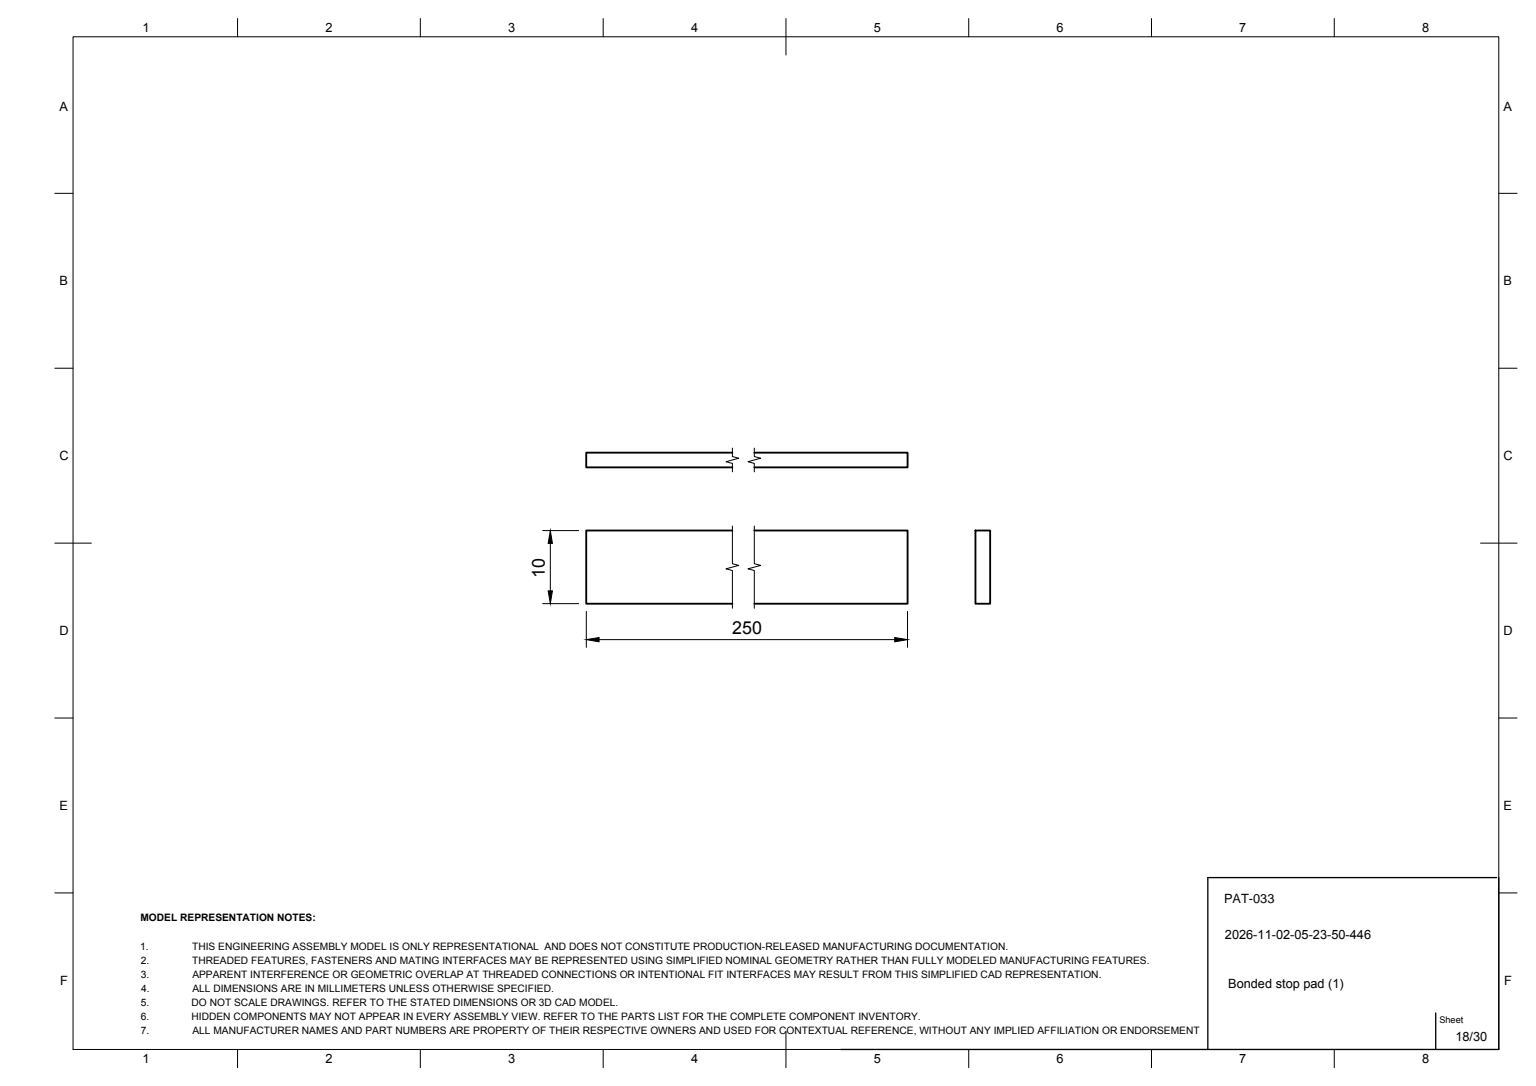
ISO-10303-21;
HEADER;
/* Generated by software containing ST-Developer
 * from STEP Tools, Inc. (www.steptools.com) 
 */

FILE_DESCRIPTION(
/* description */ ('Dual-rail gantry carriage'),
/* implementation_level */ '2;1');

FILE_NAME(
/* name */ 'Bonded stop pad (1).step',
/* time_stamp */ '2026-10-27T10:49:15-07:00',
/* author */ (''),
/* organization */ (''),
/* preprocessor_version */ 'ST-DEVELOPER v20.2',
/* originating_system */ 'Autodesk Translation Framework v15.17.0.0',
/* authorisation */ '');

FILE_SCHEMA (('AUTOMOTIVE_DESIGN { 1 0 10303 214 3 1 1 }'));
ENDSEC;

DATA;
#10=MECHANICAL_DESIGN_GEOMETRIC_PRESENTATION_REPRESENTATION('',(#598),#12804);
#536=SHAPE_REPRESENTATION_RELATIONSHIP('SRR','None',#13014,#567);
#567=ADVANCED_BREP_SHAPE_REPRESENTATION('',(#629),#12784);
#598=STYLED_ITEM('',(#13261),#629);
#629=MANIFOLD_SOLID_BREP('Body1',#7376);
#850=PLANE('',#7939);
#851=PLANE('',#7940);
#852=PLANE('',#7941);
#853=PLANE('',#7942);
#854=PLANE('',#7943);
#855=PLANE('',#7944);
#1166=FACE_OUTER_BOUND('',#1603,.T.);
#1167=FACE_OUTER_BOUND('',#1604,.T.);
#1168=FACE_OUTER_BOUND('',#1605,.T.);
#1169=FACE_OUTER_BOUND('',#1606,.T.);
#1170=FACE_OUTER_BOUND('',#1607,.T.);
#1171=FACE_OUTER_BOUND('',#1608,.T.);
#1603=EDGE_LOOP('',(#5603,#5604,#5605,#5606));
#1604=EDGE_LOOP('',(#5607,#5608,#5609,#5610));
#1605=EDGE_LOOP('',(#5611,#5612,#5613,#5614));
#1606=EDGE_LOOP('',(#5615,#5616,#5617,#5618));
#1607=EDGE_LOOP('',(#5619,#5620,#5621,#5622));
#1608=EDGE_LOOP('',(#5623,#5624,#5625,#5626));
#2152=LINE('',#11261,#2861);
#2153=LINE('',#11263,#2862);
#2154=LINE('',#11265,#2863);
#2155=LINE('',#11266,#2864);
#2156=LINE('',#11269,#2865);
#2157=LINE('',#11271,#2866);
#2158=LINE('',#11272,#2867);
#2159=LINE('',#11275,#2868);
#2160=LINE('',#11277,#2869);
#2161=LINE('',#11278,#2870);
#2162=LINE('',#11280,#2871);
#2163=LINE('',#11281,#2872);
#2861=VECTOR('',#9089,1.);
#2862=VECTOR('',#9090,1.);
#2863=VECTOR('',#9091,1.);
#2864=VECTOR('',#9092,1.);
#2865=VECTOR('',#9095,1.);
#2866=VECTOR('',#9096,1.);
#2867=VECTOR('',#9097,1.);
#2868=VECTOR('',#9100,1.);
#2869=VECTOR('',#9101,1.);
#2870=VECTOR('',#9102,1.);
#2871=VECTOR('',#9105,1.);
#2872=VECTOR('',#9106,1.);
#3734=VERTEX_POINT('',#11259);
#3735=VERTEX_POINT('',#11260);
#3736=VERTEX_POINT('',#11262);
#3737=VERTEX_POINT('',#11264);
#3738=VERTEX_POINT('',#11268);
#3739=VERTEX_POINT('',#11270);
#3740=VERTEX_POINT('',#11274);
#3741=VERTEX_POINT('',#11276);
#4424=EDGE_CURVE('',#3734,#3735,#2152,.T.);
#4425=EDGE_CURVE('',#3735,#3736,#2153,.T.);
#4426=EDGE_CURVE('',#3737,#3736,#2154,.T.);
#4427=EDGE_CURVE('',#3734,#3737,#2155,.T.);
#4428=EDGE_CURVE('',#3738,#3734,#2156,.T.);
#4429=EDGE_CURVE('',#3739,#3737,#2157,.T.);
#4430=EDGE_CURVE('',#3738,#3739,#2158,.T.);
#4431=EDGE_CURVE('',#3740,#3738,#2159,.T.);
#4432=EDGE_CURVE('',#3741,#3739,#2160,.T.);
#4433=EDGE_CURVE('',#3740,#3741,#2161,.T.);
#4434=EDGE_CURVE('',#3735,#3740,#2162,.T.);
#4435=EDGE_CURVE('',#3736,#3741,#2163,.T.);
#5603=ORIENTED_EDGE('',*,*,#4424,.T.);
#5604=ORIENTED_EDGE('',*,*,#4425,.T.);
#5605=ORIENTED_EDGE('',*,*,#4426,.F.);
#5606=ORIENTED_EDGE('',*,*,#4427,.F.);
#5607=ORIENTED_EDGE('',*,*,#4428,.T.);
#5608=ORIENTED_EDGE('',*,*,#4427,.T.);
#5609=ORIENTED_EDGE('',*,*,#4429,.F.);
#5610=ORIENTED_EDGE('',*,*,#4430,.F.);
#5611=ORIENTED_EDGE('',*,*,#4431,.T.);
#5612=ORIENTED_EDGE('',*,*,#4430,.T.);
#5613=ORIENTED_EDGE('',*,*,#4432,.F.);
#5614=ORIENTED_EDGE('',*,*,#4433,.F.);
#5615=ORIENTED_EDGE('',*,*,#4434,.T.);
#5616=ORIENTED_EDGE('',*,*,#4433,.T.);
#5617=ORIENTED_EDGE('',*,*,#4435,.F.);
#5618=ORIENTED_EDGE('',*,*,#4425,.F.);
#5619=ORIENTED_EDGE('',*,*,#4435,.T.);
#5620=ORIENTED_EDGE('',*,*,#4432,.T.);
#5621=ORIENTED_EDGE('',*,*,#4429,.T.);
#5622=ORIENTED_EDGE('',*,*,#4426,.T.);
#5623=ORIENTED_EDGE('',*,*,#4434,.F.);
#5624=ORIENTED_EDGE('',*,*,#4424,.F.);
#5625=ORIENTED_EDGE('',*,*,#4428,.F.);
#5626=ORIENTED_EDGE('',*,*,#4431,.F.);
#7092=ADVANCED_FACE('',(#1166),#850,.T.);
#7093=ADVANCED_FACE('',(#1167),#851,.T.);
#7094=ADVANCED_FACE('',(#1168),#852,.T.);
#7095=ADVANCED_FACE('',(#1169),#853,.T.);
#7096=ADVANCED_FACE('',(#1170),#854,.T.);
#7097=ADVANCED_FACE('',(#1171),#855,.F.);
#7376=CLOSED_SHELL('',(#7092,#7093,#7094,#7095,#7096,#7097));
#7938=AXIS2_PLACEMENT_3D('',#11257,#9085,#9086);
#7939=AXIS2_PLACEMENT_3D('',#11258,#9087,#9088);
#7940=AXIS2_PLACEMENT_3D('',#11267,#9093,#9094);
#7941=AXIS2_PLACEMENT_3D('',#11273,#9098,#9099);
#7942=AXIS2_PLACEMENT_3D('',#11279,#9103,#9104);
#7943=AXIS2_PLACEMENT_3D('',#11282,#9107,#9108);
#7944=AXIS2_PLACEMENT_3D('',#11283,#9109,#9110);
#9085=DIRECTION('axis',(0.,0.,1.));
#9086=DIRECTION('refdir',(1.,0.,0.));
#9087=DIRECTION('center_axis',(0.,1.,0.));
#9088=DIRECTION('ref_axis',(-1.,0.,0.));
#9089=DIRECTION('',(-1.,0.,0.));
#9090=DIRECTION('',(0.,0.,1.));
#9091=DIRECTION('',(-1.,0.,0.));
#9092=DIRECTION('',(0.,0.,1.));
#9093=DIRECTION('center_axis',(1.,0.,0.));
#9094=DIRECTION('ref_axis',(0.,1.,0.));
#9095=DIRECTION('',(0.,1.,0.));
#9096=DIRECTION('',(0.,1.,0.));
#9097=DIRECTION('',(0.,0.,1.));
#9098=DIRECTION('center_axis',(0.,-1.,0.));
#9099=DIRECTION('ref_axis',(1.,0.,0.));
#9100=DIRECTION('',(1.,0.,0.));
#9101=DIRECTION('',(1.,0.,0.));
#9102=DIRECTION('',(0.,0.,1.));
#9103=DIRECTION('center_axis',(-1.,0.,0.));
#9104=DIRECTION('ref_axis',(0.,-1.,0.));
#9105=DIRECTION('',(0.,-1.,0.));
#9106=DIRECTION('',(0.,-1.,0.));
#9107=DIRECTION('center_axis',(0.,0.,1.));
#9108=DIRECTION('ref_axis',(1.,0.,0.));
#9109=DIRECTION('center_axis',(0.,0.,1.));
#9110=DIRECTION('ref_axis',(1.,0.,0.));
#11257=CARTESIAN_POINT('',(0.,0.,0.));
#11258=CARTESIAN_POINT('Origin',(32.,12.5,5.2));
#11259=CARTESIAN_POINT('',(32.,12.5,5.2));
#11260=CARTESIAN_POINT('',(31.8,12.5,5.2));
#11261=CARTESIAN_POINT('',(32.,12.5,5.2));
#11262=CARTESIAN_POINT('',(31.8,12.5,6.2));
#11263=CARTESIAN_POINT('',(31.8,12.5,5.2));
#11264=CARTESIAN_POINT('',(32.,12.5,6.2));
#11265=CARTESIAN_POINT('',(32.,12.5,6.2));
#11266=CARTESIAN_POINT('',(32.,12.5,5.2));
#11267=CARTESIAN_POINT('Origin',(32.,-12.5,5.2));
#11268=CARTESIAN_POINT('',(32.,-12.5,5.2));
#11269=CARTESIAN_POINT('',(32.,-12.5,5.2));
#11270=CARTESIAN_POINT('',(32.,-12.5,6.2));
#11271=CARTESIAN_POINT('',(32.,-12.5,6.2));
#11272=CARTESIAN_POINT('',(32.,-12.5,5.2));
#11273=CARTESIAN_POINT('Origin',(31.8,-12.5,5.2));
#11274=CARTESIAN_POINT('',(31.8,-12.5,5.2));
#11275=CARTESIAN_POINT('',(31.8,-12.5,5.2));
#11276=CARTESIAN_POINT('',(31.8,-12.5,6.2));
#11277=CARTESIAN_POINT('',(31.8,-12.5,6.2));
#11278=CARTESIAN_POINT('',(31.8,-12.5,5.2));
#11279=CARTESIAN_POINT('Origin',(31.8,12.5,5.2));
#11280=CARTESIAN_POINT('',(31.8,12.5,5.2));
#11281=CARTESIAN_POINT('',(31.8,12.5,6.2));
#11282=CARTESIAN_POINT('Origin',(31.9,0.,6.2));
#11283=CARTESIAN_POINT('Origin',(31.9,0.,5.2));
#12748=UNCERTAINTY_MEASURE_WITH_UNIT(LENGTH_MEASURE(0.001),#12805,
'DISTANCE_ACCURACY_VALUE',
'Maximum model space distance between geometric entities at asserted c
onnectivities');
#12768=UNCERTAINTY_MEASURE_WITH_UNIT(LENGTH_MEASURE(0.001),#12805,
'DISTANCE_ACCURACY_VALUE',
'Maximum model space distance between geometric entities at asserted c
onnectivities');
#12784=(
GEOMETRIC_REPRESENTATION_CONTEXT(3)
GLOBAL_UNCERTAINTY_ASSIGNED_CONTEXT((#12748))
GLOBAL_UNIT_ASSIGNED_CONTEXT((#12805,#12807,#12808))
REPRESENTATION_CONTEXT('','3D')
);
#12804=(
GEOMETRIC_REPRESENTATION_CONTEXT(3)
GLOBAL_UNCERTAINTY_ASSIGNED_CONTEXT((#12768))
GLOBAL_UNIT_ASSIGNED_CONTEXT((#12805,#12807,#12808))
REPRESENTATION_CONTEXT('','3D')
);
#12805=(
LENGTH_UNIT()
NAMED_UNIT(*)
SI_UNIT(.CENTI.,.METRE.)
);
#12807=(
NAMED_UNIT(*)
PLANE_ANGLE_UNIT()
SI_UNIT($,.RADIAN.)
);
#12808=(
NAMED_UNIT(*)
SI_UNIT($,.STERADIAN.)
SOLID_ANGLE_UNIT()
);
#12824=SHAPE_DEFINITION_REPRESENTATION(#12859,#13014);
#12859=PRODUCT_DEFINITION_SHAPE('',$,#13050);
#13014=SHAPE_REPRESENTATION('',(#7938),#12784);
#13034=PRODUCT_DEFINITION_CONTEXT('part definition',#13141,'design');
#13050=PRODUCT_DEFINITION('Bonded stop pad (1)','Bonded stop pad (1)',#13085,
#13034);
#13085=PRODUCT_DEFINITION_FORMATION('',$,#13158);
#13141=APPLICATION_CONTEXT(
'Core Data for Automotive Mechanical Design Process');
#13142=PRODUCT_CONTEXT('part definition',#13141,'mechanical');
#13158=PRODUCT('Bonded stop pad (1)','Bonded stop pad (1)',
'Bonded stop pad (1)',(#13142));
#13255=COLOUR_RGB('Off White',0.89,0.88,0.83);
#13256=FILL_AREA_STYLE_COLOUR('',#13255);
#13257=FILL_AREA_STYLE('',(#13256));
#13258=SURFACE_STYLE_FILL_AREA(#13257);
#13259=SURFACE_SIDE_STYLE('',(#13258));
#13260=SURFACE_STYLE_USAGE(.BOTH.,#13259);
#13261=PRESENTATION_STYLE_ASSIGNMENT((#13260));
ENDSEC;
END-ISO-10303-21;
